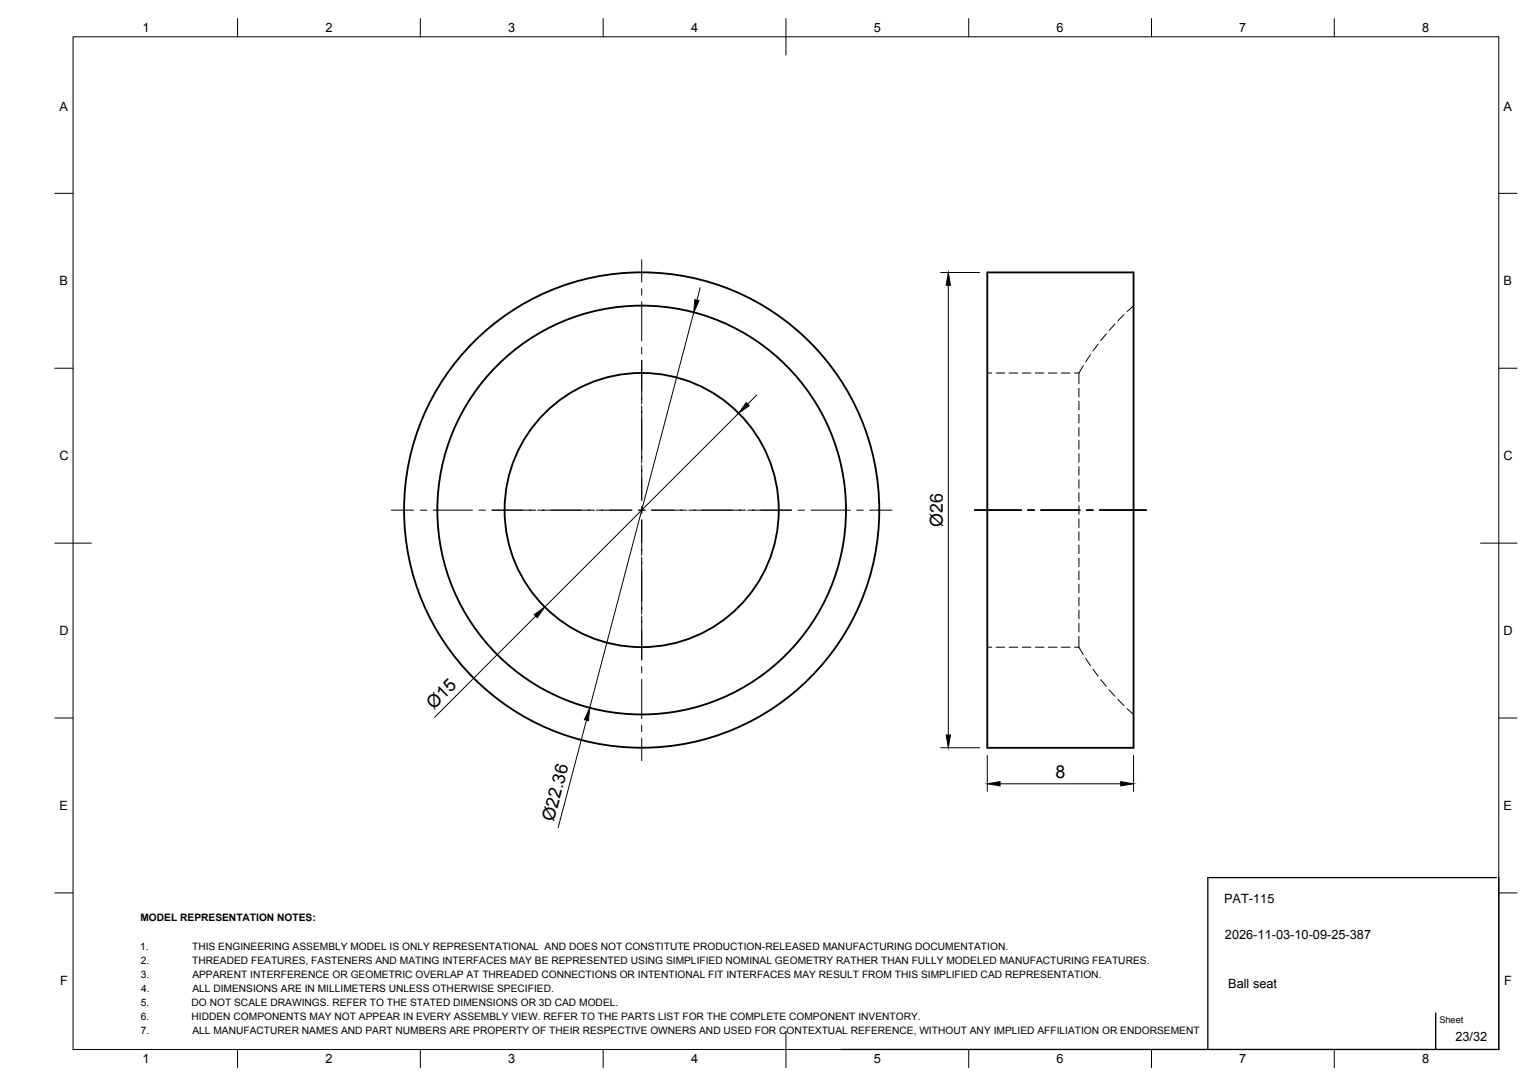
ISO-10303-21;
HEADER;
/* Generated by software containing ST-Developer
 * from STEP Tools, Inc. (www.steptools.com) 
 */

FILE_DESCRIPTION(
/* description */ ('Union bypass pipe loop'),
/* implementation_level */ '2;1');

FILE_NAME(
/* name */ 'Ball seat.step',
/* time_stamp */ '2026-10-27T21:00:29-07:00',
/* author */ (''),
/* organization */ (''),
/* preprocessor_version */ 'ST-DEVELOPER v20.2',
/* originating_system */ 'Autodesk Translation Framework v15.17.0.0',
/* authorisation */ '');

FILE_SCHEMA (('AUTOMOTIVE_DESIGN { 1 0 10303 214 3 1 1 }'));
ENDSEC;

DATA;
#10=MECHANICAL_DESIGN_GEOMETRIC_PRESENTATION_REPRESENTATION('',(#452),#10095);
#388=SHAPE_REPRESENTATION_RELATIONSHIP('SRR','None',#10257,#420);
#420=ADVANCED_BREP_SHAPE_REPRESENTATION('',(#484),#10069);
#452=STYLED_ITEM('',(#10486),#484);
#484=MANIFOLD_SOLID_BREP('Body1',#5523);
#507=SPHERICAL_SURFACE('',#6082,1.5);
#565=FACE_BOUND('',#1308,.T.);
#566=FACE_BOUND('',#1312,.T.);
#567=FACE_BOUND('',#1314,.T.);
#682=PLANE('',#6090);
#683=PLANE('',#6091);
#921=FACE_OUTER_BOUND('',#1307,.T.);
#922=FACE_OUTER_BOUND('',#1309,.T.);
#923=FACE_OUTER_BOUND('',#1310,.T.);
#924=FACE_OUTER_BOUND('',#1311,.T.);
#925=FACE_OUTER_BOUND('',#1313,.T.);
#1307=EDGE_LOOP('',(#4112));
#1308=EDGE_LOOP('',(#4113));
#1309=EDGE_LOOP('',(#4114,#4115,#4116,#4117));
#1310=EDGE_LOOP('',(#4118,#4119,#4120,#4121));
#1311=EDGE_LOOP('',(#4122));
#1312=EDGE_LOOP('',(#4123));
#1313=EDGE_LOOP('',(#4124));
#1314=EDGE_LOOP('',(#4125));
#1730=LINE('',#8839,#2106);
#1731=LINE('',#8845,#2107);
#2106=VECTOR('',#7088,0.75);
#2107=VECTOR('',#7095,1.3);
#2455=CIRCLE('',#6083,1.11803398874989);
#2456=CIRCLE('',#6084,0.75);
#2457=CIRCLE('',#6086,0.75);
#2458=CIRCLE('',#6088,1.3);
#2459=CIRCLE('',#6089,1.3);
#2755=VERTEX_POINT('',#8833);
#2756=VERTEX_POINT('',#8835);
#2757=VERTEX_POINT('',#8838);
#2758=VERTEX_POINT('',#8842);
#2759=VERTEX_POINT('',#8844);
#3254=EDGE_CURVE('',#2755,#2755,#2455,.T.);
#3255=EDGE_CURVE('',#2756,#2756,#2456,.T.);
#3256=EDGE_CURVE('',#2756,#2757,#1730,.T.);
#3257=EDGE_CURVE('',#2757,#2757,#2457,.T.);
#3258=EDGE_CURVE('',#2758,#2758,#2458,.T.);
#3259=EDGE_CURVE('',#2758,#2759,#1731,.T.);
#3260=EDGE_CURVE('',#2759,#2759,#2459,.T.);
#4112=ORIENTED_EDGE('',*,*,#3254,.F.);
#4113=ORIENTED_EDGE('',*,*,#3255,.F.);
#4114=ORIENTED_EDGE('',*,*,#3255,.T.);
#4115=ORIENTED_EDGE('',*,*,#3256,.T.);
#4116=ORIENTED_EDGE('',*,*,#3257,.T.);
#4117=ORIENTED_EDGE('',*,*,#3256,.F.);
#4118=ORIENTED_EDGE('',*,*,#3258,.F.);
#4119=ORIENTED_EDGE('',*,*,#3259,.T.);
#4120=ORIENTED_EDGE('',*,*,#3260,.T.);
#4121=ORIENTED_EDGE('',*,*,#3259,.F.);
#4122=ORIENTED_EDGE('',*,*,#3258,.T.);
#4123=ORIENTED_EDGE('',*,*,#3254,.T.);
#4124=ORIENTED_EDGE('',*,*,#3260,.F.);
#4125=ORIENTED_EDGE('',*,*,#3257,.F.);
#5116=CYLINDRICAL_SURFACE('',#6085,0.75);
#5117=CYLINDRICAL_SURFACE('',#6087,1.3);
#5270=ADVANCED_FACE('',(#921,#565),#507,.F.);
#5271=ADVANCED_FACE('',(#922),#5116,.F.);
#5272=ADVANCED_FACE('',(#923),#5117,.T.);
#5273=ADVANCED_FACE('',(#924,#566),#682,.T.);
#5274=ADVANCED_FACE('',(#925,#567),#683,.F.);
#5523=CLOSED_SHELL('',(#5270,#5271,#5272,#5273,#5274));
#6081=AXIS2_PLACEMENT_3D('',#8831,#7078,#7079);
#6082=AXIS2_PLACEMENT_3D('',#8832,#7080,#7081);
#6083=AXIS2_PLACEMENT_3D('',#8834,#7082,#7083);
#6084=AXIS2_PLACEMENT_3D('',#8836,#7084,#7085);
#6085=AXIS2_PLACEMENT_3D('',#8837,#7086,#7087);
#6086=AXIS2_PLACEMENT_3D('',#8840,#7089,#7090);
#6087=AXIS2_PLACEMENT_3D('',#8841,#7091,#7092);
#6088=AXIS2_PLACEMENT_3D('',#8843,#7093,#7094);
#6089=AXIS2_PLACEMENT_3D('',#8846,#7096,#7097);
#6090=AXIS2_PLACEMENT_3D('',#8847,#7098,#7099);
#6091=AXIS2_PLACEMENT_3D('',#8848,#7100,#7101);
#7078=DIRECTION('axis',(0.,0.,1.));
#7079=DIRECTION('refdir',(1.,0.,0.));
#7080=DIRECTION('center_axis',(6.12323399573677E-17,0.,1.));
#7081=DIRECTION('ref_axis',(1.,0.,0.));
#7082=DIRECTION('center_axis',(0.,-1.,0.));
#7083=DIRECTION('ref_axis',(0.,0.,-1.));
#7084=DIRECTION('center_axis',(0.,1.,0.));
#7085=DIRECTION('ref_axis',(1.,0.,0.));
#7086=DIRECTION('center_axis',(0.,1.,0.));
#7087=DIRECTION('ref_axis',(1.,0.,0.));
#7088=DIRECTION('',(0.,-1.,0.));
#7089=DIRECTION('center_axis',(0.,-1.,0.));
#7090=DIRECTION('ref_axis',(1.,0.,0.));
#7091=DIRECTION('center_axis',(0.,1.,0.));
#7092=DIRECTION('ref_axis',(1.,0.,0.));
#7093=DIRECTION('center_axis',(0.,1.,0.));
#7094=DIRECTION('ref_axis',(1.,0.,0.));
#7095=DIRECTION('',(0.,-1.,0.));
#7096=DIRECTION('center_axis',(0.,1.,0.));
#7097=DIRECTION('ref_axis',(1.,0.,0.));
#7098=DIRECTION('center_axis',(0.,1.,0.));
#7099=DIRECTION('ref_axis',(1.,0.,0.));
#7100=DIRECTION('center_axis',(0.,1.,0.));
#7101=DIRECTION('ref_axis',(1.,0.,0.));
#8831=CARTESIAN_POINT('',(0.,0.,0.));
#8832=CARTESIAN_POINT('Origin',(0.,0.,5.));
#8833=CARTESIAN_POINT('',(-1.36919674566051E-16,-1.,6.11803398874989));
#8834=CARTESIAN_POINT('Origin',(0.,-1.,5.));
#8835=CARTESIAN_POINT('',(-0.75,-1.29903810567666,5.));
#8836=CARTESIAN_POINT('Origin',(0.,-1.29903810567666,5.));
#8837=CARTESIAN_POINT('Origin',(0.,-1.8,5.));
#8838=CARTESIAN_POINT('',(-0.75,-1.8,5.));
#8839=CARTESIAN_POINT('',(-0.75,-1.8,5.));
#8840=CARTESIAN_POINT('Origin',(0.,-1.8,5.));
#8841=CARTESIAN_POINT('Origin',(0.,-1.8,5.));
#8842=CARTESIAN_POINT('',(-1.3,-1.,5.));
#8843=CARTESIAN_POINT('Origin',(0.,-1.,5.));
#8844=CARTESIAN_POINT('',(-1.3,-1.8,5.));
#8845=CARTESIAN_POINT('',(-1.3,-1.8,5.));
#8846=CARTESIAN_POINT('Origin',(0.,-1.8,5.));
#8847=CARTESIAN_POINT('Origin',(0.,-1.,5.));
#8848=CARTESIAN_POINT('Origin',(0.,-1.8,5.));
#10032=UNCERTAINTY_MEASURE_WITH_UNIT(LENGTH_MEASURE(0.001),#10096,
'DISTANCE_ACCURACY_VALUE',
'Maximum model space distance between geometric entities at asserted c
onnectivities');
#10058=UNCERTAINTY_MEASURE_WITH_UNIT(LENGTH_MEASURE(0.001),#10096,
'DISTANCE_ACCURACY_VALUE',
'Maximum model space distance between geometric entities at asserted c
onnectivities');
#10069=(
GEOMETRIC_REPRESENTATION_CONTEXT(3)
GLOBAL_UNCERTAINTY_ASSIGNED_CONTEXT((#10032))
GLOBAL_UNIT_ASSIGNED_CONTEXT((#10096,#10098,#10099))
REPRESENTATION_CONTEXT('','3D')
);
#10095=(
GEOMETRIC_REPRESENTATION_CONTEXT(3)
GLOBAL_UNCERTAINTY_ASSIGNED_CONTEXT((#10058))
GLOBAL_UNIT_ASSIGNED_CONTEXT((#10096,#10098,#10099))
REPRESENTATION_CONTEXT('','3D')
);
#10096=(
LENGTH_UNIT()
NAMED_UNIT(*)
SI_UNIT(.CENTI.,.METRE.)
);
#10098=(
NAMED_UNIT(*)
PLANE_ANGLE_UNIT()
SI_UNIT($,.RADIAN.)
);
#10099=(
NAMED_UNIT(*)
SI_UNIT($,.STERADIAN.)
SOLID_ANGLE_UNIT()
);
#10110=SHAPE_DEFINITION_REPRESENTATION(#10146,#10257);
#10146=PRODUCT_DEFINITION_SHAPE('',$,#10294);
#10257=SHAPE_REPRESENTATION('',(#6081),#10069);
#10283=PRODUCT_DEFINITION_CONTEXT('part definition',#10393,'design');
#10294=PRODUCT_DEFINITION('Ball seat','Ball seat',#10330,#10283);
#10330=PRODUCT_DEFINITION_FORMATION('',$,#10405);
#10393=APPLICATION_CONTEXT(
'Core Data for Automotive Mechanical Design Process');
#10394=PRODUCT_CONTEXT('part definition',#10393,'mechanical');
#10405=PRODUCT('Ball seat','Ball seat','Ball seat',(#10394));
#10480=COLOUR_RGB('Light Blue',0.38,0.62,0.78);
#10481=FILL_AREA_STYLE_COLOUR('',#10480);
#10482=FILL_AREA_STYLE('',(#10481));
#10483=SURFACE_STYLE_FILL_AREA(#10482);
#10484=SURFACE_SIDE_STYLE('',(#10483));
#10485=SURFACE_STYLE_USAGE(.BOTH.,#10484);
#10486=PRESENTATION_STYLE_ASSIGNMENT((#10485));
ENDSEC;
END-ISO-10303-21;
